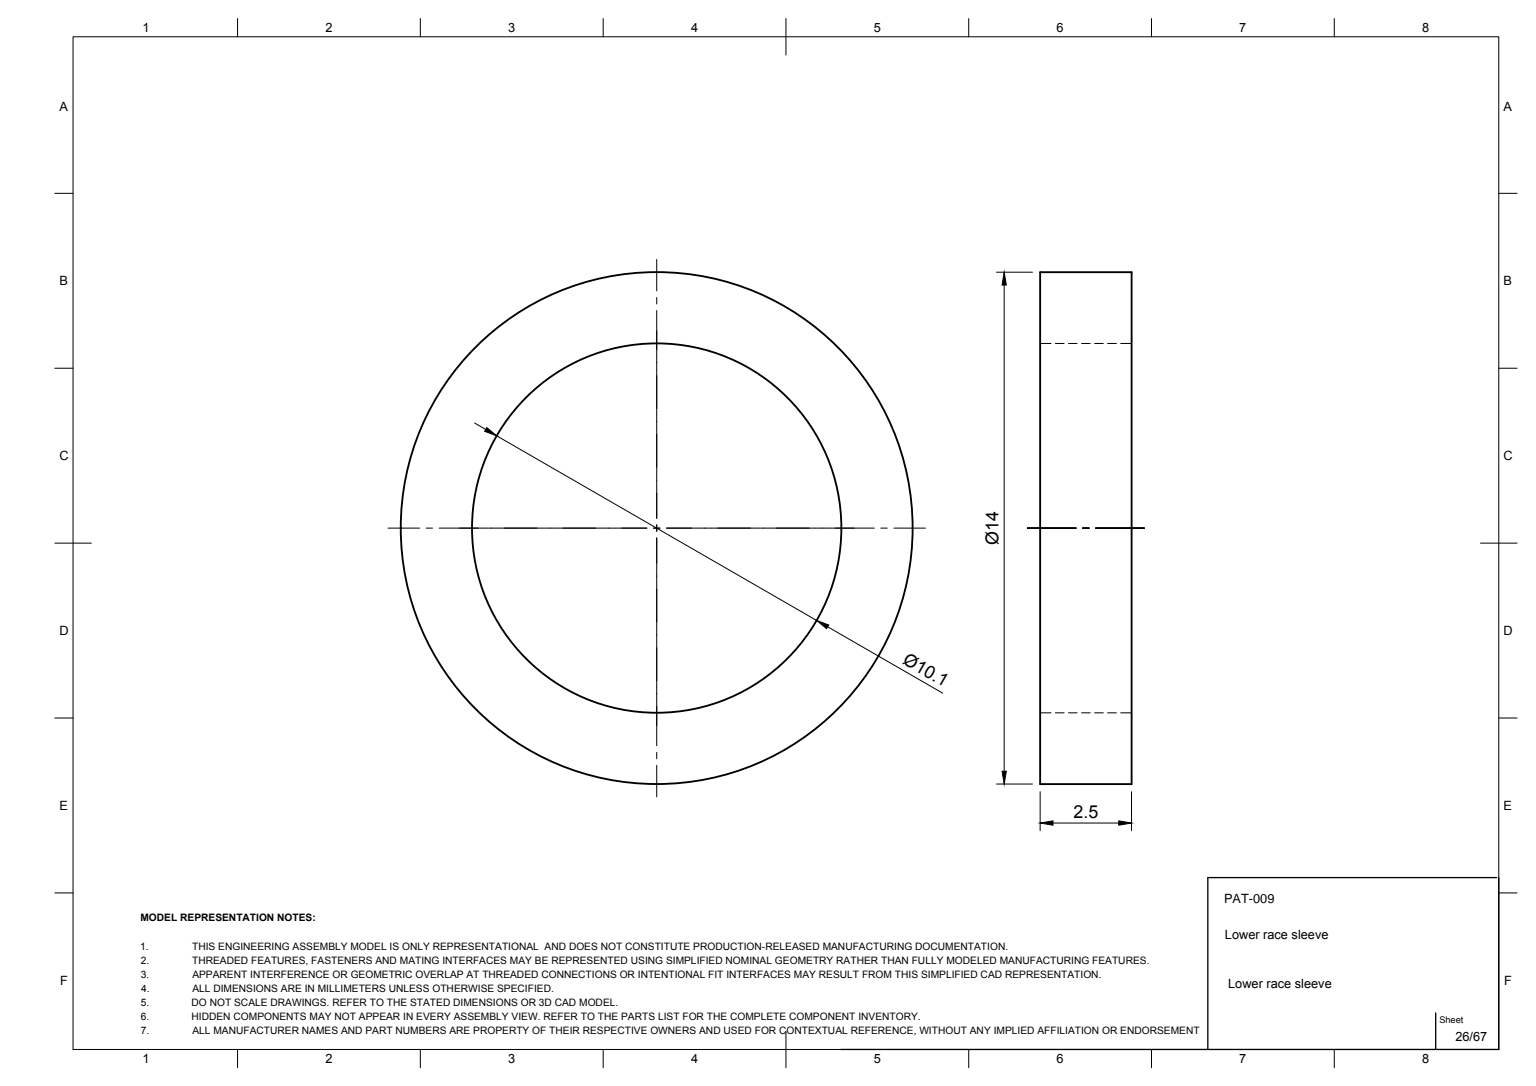
ISO-10303-21;
HEADER;
/* Generated by software containing ST-Developer
 * from STEP Tools, Inc. (www.steptools.com) 
 */

FILE_DESCRIPTION(
/* description */ ('Bell-crank linkage with push rods'),
/* implementation_level */ '2;1');

FILE_NAME(
/* name */ 'Lower race sleeve.step',
/* time_stamp */ '2026-10-28T03:25:15-07:00',
/* author */ (''),
/* organization */ (''),
/* preprocessor_version */ 'ST-DEVELOPER v20.2',
/* originating_system */ 'Autodesk Translation Framework v15.17.0.0',
/* authorisation */ '');

FILE_SCHEMA (('AUTOMOTIVE_DESIGN { 1 0 10303 214 3 1 1 }'));
ENDSEC;

DATA;
#10=MECHANICAL_DESIGN_GEOMETRIC_PRESENTATION_REPRESENTATION('',(#631),#16678);
#515=SHAPE_REPRESENTATION_RELATIONSHIP('SRR','None',#16933,#569);
#569=ADVANCED_BREP_SHAPE_REPRESENTATION('',(#692),#16638);
#631=STYLED_ITEM('',(#17277),#692);
#692=MANIFOLD_SOLID_BREP('Body1',#8822);
#832=FACE_BOUND('',#2135,.T.);
#833=FACE_BOUND('',#2137,.T.);
#1095=PLANE('',#10009);
#1096=PLANE('',#10010);
#1503=FACE_OUTER_BOUND('',#2132,.T.);
#1504=FACE_OUTER_BOUND('',#2133,.T.);
#1505=FACE_OUTER_BOUND('',#2134,.T.);
#1506=FACE_OUTER_BOUND('',#2136,.T.);
#2132=EDGE_LOOP('',(#7061,#7062,#7063,#7064));
#2133=EDGE_LOOP('',(#7065,#7066,#7067,#7068));
#2134=EDGE_LOOP('',(#7069));
#2135=EDGE_LOOP('',(#7070));
#2136=EDGE_LOOP('',(#7071));
#2137=EDGE_LOOP('',(#7072));
#2809=LINE('',#15257,#3358);
#2810=LINE('',#15263,#3359);
#3358=VECTOR('',#12009,0.505);
#3359=VECTOR('',#12016,0.7);
#3894=CIRCLE('',#10004,0.505);
#3895=CIRCLE('',#10005,0.505);
#3896=CIRCLE('',#10007,0.7);
#3897=CIRCLE('',#10008,0.7);
#4500=VERTEX_POINT('',#15254);
#4501=VERTEX_POINT('',#15256);
#4502=VERTEX_POINT('',#15260);
#4503=VERTEX_POINT('',#15262);
#5408=EDGE_CURVE('',#4500,#4500,#3894,.T.);
#5409=EDGE_CURVE('',#4500,#4501,#2809,.T.);
#5410=EDGE_CURVE('',#4501,#4501,#3895,.T.);
#5411=EDGE_CURVE('',#4502,#4502,#3896,.T.);
#5412=EDGE_CURVE('',#4502,#4503,#2810,.T.);
#5413=EDGE_CURVE('',#4503,#4503,#3897,.T.);
#7061=ORIENTED_EDGE('',*,*,#5408,.F.);
#7062=ORIENTED_EDGE('',*,*,#5409,.T.);
#7063=ORIENTED_EDGE('',*,*,#5410,.T.);
#7064=ORIENTED_EDGE('',*,*,#5409,.F.);
#7065=ORIENTED_EDGE('',*,*,#5411,.F.);
#7066=ORIENTED_EDGE('',*,*,#5412,.T.);
#7067=ORIENTED_EDGE('',*,*,#5413,.T.);
#7068=ORIENTED_EDGE('',*,*,#5412,.F.);
#7069=ORIENTED_EDGE('',*,*,#5411,.T.);
#7070=ORIENTED_EDGE('',*,*,#5408,.T.);
#7071=ORIENTED_EDGE('',*,*,#5413,.F.);
#7072=ORIENTED_EDGE('',*,*,#5410,.F.);
#8166=CYLINDRICAL_SURFACE('',#10003,0.505);
#8167=CYLINDRICAL_SURFACE('',#10006,0.7);
#8528=ADVANCED_FACE('',(#1503),#8166,.F.);
#8529=ADVANCED_FACE('',(#1504),#8167,.T.);
#8530=ADVANCED_FACE('',(#1505,#832),#1095,.T.);
#8531=ADVANCED_FACE('',(#1506,#833),#1096,.F.);
#8822=CLOSED_SHELL('',(#8528,#8529,#8530,#8531));
#10002=AXIS2_PLACEMENT_3D('',#15252,#12003,#12004);
#10003=AXIS2_PLACEMENT_3D('',#15253,#12005,#12006);
#10004=AXIS2_PLACEMENT_3D('',#15255,#12007,#12008);
#10005=AXIS2_PLACEMENT_3D('',#15258,#12010,#12011);
#10006=AXIS2_PLACEMENT_3D('',#15259,#12012,#12013);
#10007=AXIS2_PLACEMENT_3D('',#15261,#12014,#12015);
#10008=AXIS2_PLACEMENT_3D('',#15264,#12017,#12018);
#10009=AXIS2_PLACEMENT_3D('',#15265,#12019,#12020);
#10010=AXIS2_PLACEMENT_3D('',#15266,#12021,#12022);
#12003=DIRECTION('axis',(0.,0.,1.));
#12004=DIRECTION('refdir',(1.,0.,0.));
#12005=DIRECTION('center_axis',(0.,0.,1.));
#12006=DIRECTION('ref_axis',(1.,0.,0.));
#12007=DIRECTION('center_axis',(0.,0.,-1.));
#12008=DIRECTION('ref_axis',(1.,0.,0.));
#12009=DIRECTION('',(0.,0.,-1.));
#12010=DIRECTION('center_axis',(0.,0.,-1.));
#12011=DIRECTION('ref_axis',(1.,0.,0.));
#12012=DIRECTION('center_axis',(0.,0.,1.));
#12013=DIRECTION('ref_axis',(1.,0.,0.));
#12014=DIRECTION('center_axis',(0.,0.,1.));
#12015=DIRECTION('ref_axis',(1.,0.,0.));
#12016=DIRECTION('',(0.,0.,-1.));
#12017=DIRECTION('center_axis',(0.,0.,1.));
#12018=DIRECTION('ref_axis',(1.,0.,0.));
#12019=DIRECTION('center_axis',(0.,0.,1.));
#12020=DIRECTION('ref_axis',(1.,0.,0.));
#12021=DIRECTION('center_axis',(0.,0.,1.));
#12022=DIRECTION('ref_axis',(1.,0.,0.));
#15252=CARTESIAN_POINT('',(0.,0.,0.));
#15253=CARTESIAN_POINT('Origin',(0.,0.,1.8));
#15254=CARTESIAN_POINT('',(-0.505,-6.18446633569413E-17,2.05));
#15255=CARTESIAN_POINT('Origin',(0.,0.,2.05));
#15256=CARTESIAN_POINT('',(-0.505,-6.18446633569413E-17,1.8));
#15257=CARTESIAN_POINT('',(-0.505,-6.18446633569413E-17,1.8));
#15258=CARTESIAN_POINT('Origin',(0.,0.,1.8));
#15259=CARTESIAN_POINT('Origin',(0.,0.,1.8));
#15260=CARTESIAN_POINT('',(-0.7,-8.57252759403147E-17,2.05));
#15261=CARTESIAN_POINT('Origin',(0.,0.,2.05));
#15262=CARTESIAN_POINT('',(-0.7,-8.57252759403147E-17,1.8));
#15263=CARTESIAN_POINT('',(-0.7,-8.57252759403147E-17,1.8));
#15264=CARTESIAN_POINT('Origin',(0.,0.,1.8));
#15265=CARTESIAN_POINT('Origin',(0.,0.,2.05));
#15266=CARTESIAN_POINT('Origin',(0.,0.,1.8));
#16574=UNCERTAINTY_MEASURE_WITH_UNIT(LENGTH_MEASURE(0.001),#16679,
'DISTANCE_ACCURACY_VALUE',
'Maximum model space distance between geometric entities at asserted c
onnectivities');
#16614=UNCERTAINTY_MEASURE_WITH_UNIT(LENGTH_MEASURE(0.001),#16679,
'DISTANCE_ACCURACY_VALUE',
'Maximum model space distance between geometric entities at asserted c
onnectivities');
#16638=(
GEOMETRIC_REPRESENTATION_CONTEXT(3)
GLOBAL_UNCERTAINTY_ASSIGNED_CONTEXT((#16574))
GLOBAL_UNIT_ASSIGNED_CONTEXT((#16679,#16681,#16682))
REPRESENTATION_CONTEXT('','3D')
);
#16678=(
GEOMETRIC_REPRESENTATION_CONTEXT(3)
GLOBAL_UNCERTAINTY_ASSIGNED_CONTEXT((#16614))
GLOBAL_UNIT_ASSIGNED_CONTEXT((#16679,#16681,#16682))
REPRESENTATION_CONTEXT('','3D')
);
#16679=(
LENGTH_UNIT()
NAMED_UNIT(*)
SI_UNIT(.CENTI.,.METRE.)
);
#16681=(
NAMED_UNIT(*)
PLANE_ANGLE_UNIT()
SI_UNIT($,.RADIAN.)
);
#16682=(
NAMED_UNIT(*)
SI_UNIT($,.STERADIAN.)
SOLID_ANGLE_UNIT()
);
#16706=SHAPE_DEFINITION_REPRESENTATION(#16774,#16933);
#16774=PRODUCT_DEFINITION_SHAPE('',$,#16997);
#16933=SHAPE_REPRESENTATION('',(#10002),#16638);
#16973=PRODUCT_DEFINITION_CONTEXT('part definition',#17164,'design');
#16997=PRODUCT_DEFINITION('Lower race sleeve','Lower race sleeve',#17060,
#16973);
#17060=PRODUCT_DEFINITION_FORMATION('',$,#17189);
#17164=APPLICATION_CONTEXT(
'Core Data for Automotive Mechanical Design Process');
#17165=PRODUCT_CONTEXT('part definition',#17164,'mechanical');
#17189=PRODUCT('Lower race sleeve','Lower race sleeve',
'Lower race sleeve',(#17165));
#17271=COLOUR_RGB('Light Blue',0.38,0.62,0.78);
#17272=FILL_AREA_STYLE_COLOUR('',#17271);
#17273=FILL_AREA_STYLE('',(#17272));
#17274=SURFACE_STYLE_FILL_AREA(#17273);
#17275=SURFACE_SIDE_STYLE('',(#17274));
#17276=SURFACE_STYLE_USAGE(.BOTH.,#17275);
#17277=PRESENTATION_STYLE_ASSIGNMENT((#17276));
ENDSEC;
END-ISO-10303-21;
